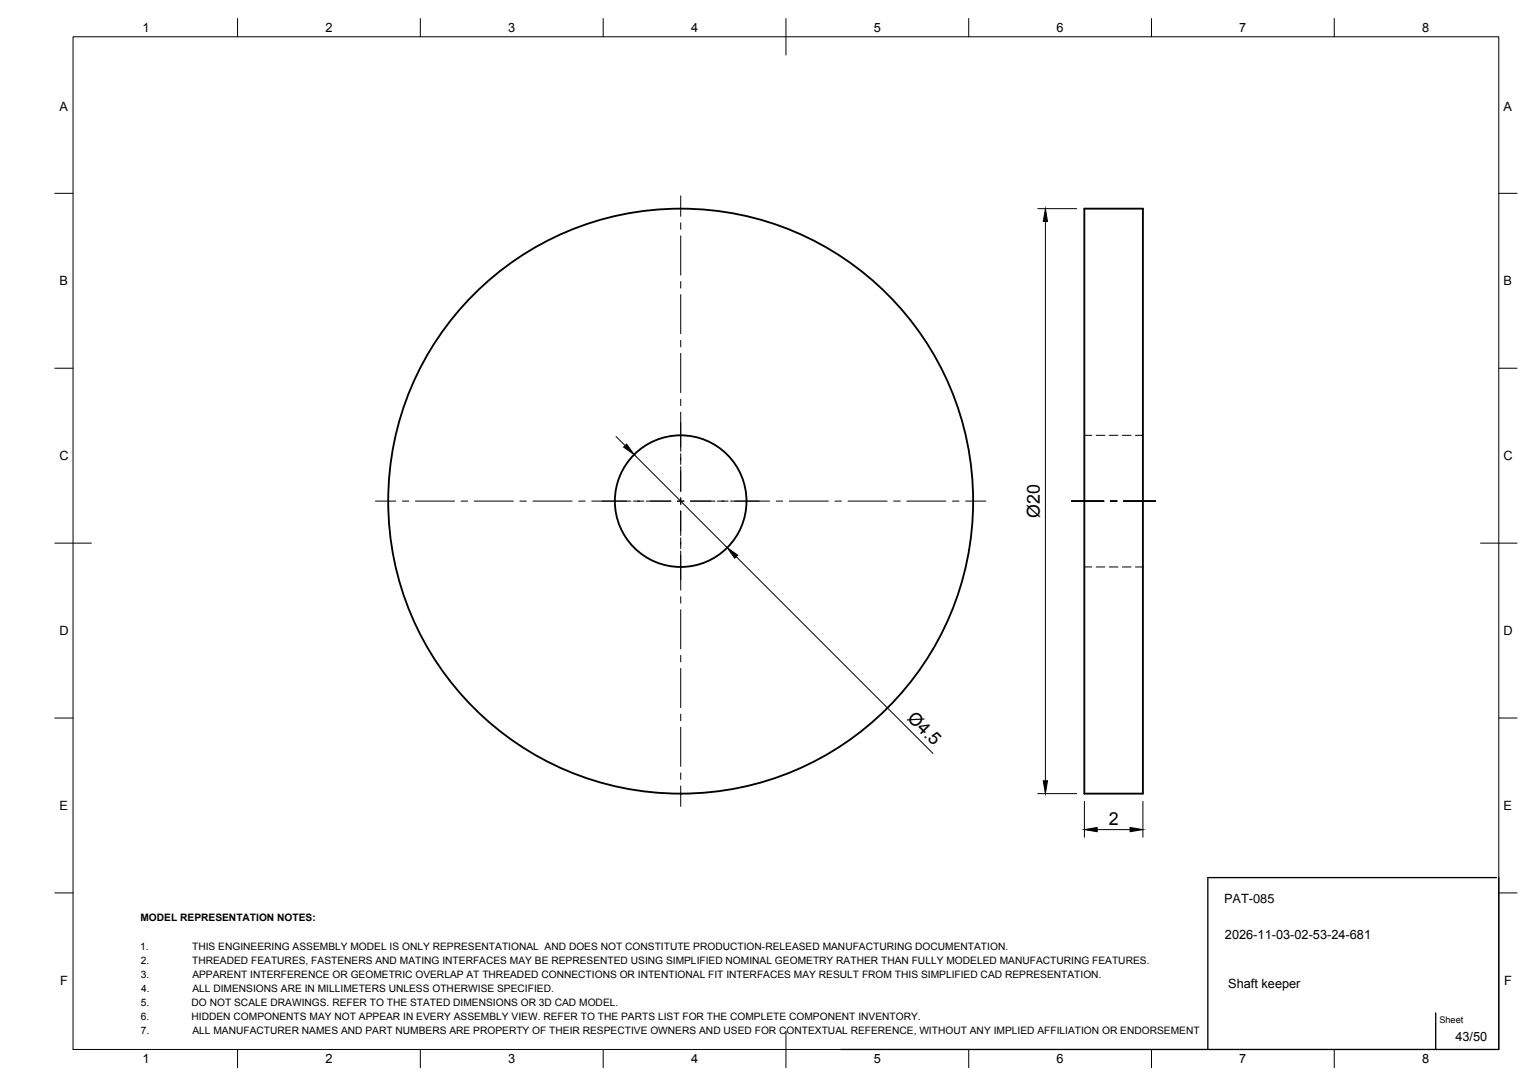
ISO-10303-21;
HEADER;
/* Generated by software containing ST-Developer
 * from STEP Tools, Inc. (www.steptools.com) 
 */

FILE_DESCRIPTION(
/* description */ ('Rack and pinion manual slide'),
/* implementation_level */ '2;1');

FILE_NAME(
/* name */ 'Shaft keeper.step',
/* time_stamp */ '2026-10-28T03:22:49-07:00',
/* author */ (''),
/* organization */ (''),
/* preprocessor_version */ 'ST-DEVELOPER v20.2',
/* originating_system */ 'Autodesk Translation Framework v15.17.0.0',
/* authorisation */ '');

FILE_SCHEMA (('AUTOMOTIVE_DESIGN { 1 0 10303 214 3 1 1 }'));
ENDSEC;

DATA;
#10=MECHANICAL_DESIGN_GEOMETRIC_PRESENTATION_REPRESENTATION('',(#774),#34851);
#675=SHAPE_REPRESENTATION_RELATIONSHIP('SRR','None',#35114,#721);
#721=ADVANCED_BREP_SHAPE_REPRESENTATION('',(#824),#34839);
#774=STYLED_ITEM('',(#35411),#824);
#824=MANIFOLD_SOLID_BREP('Body1',#13797);
#1022=FACE_BOUND('',#3036,.T.);
#1023=FACE_BOUND('',#3038,.T.);
#1456=PLANE('',#15269);
#1457=PLANE('',#15270);
#2105=FACE_OUTER_BOUND('',#3033,.T.);
#2106=FACE_OUTER_BOUND('',#3034,.T.);
#2107=FACE_OUTER_BOUND('',#3035,.T.);
#2108=FACE_OUTER_BOUND('',#3037,.T.);
#3033=EDGE_LOOP('',(#12026,#12027,#12028,#12029));
#3034=EDGE_LOOP('',(#12030,#12031,#12032,#12033));
#3035=EDGE_LOOP('',(#12034));
#3036=EDGE_LOOP('',(#12035));
#3037=EDGE_LOOP('',(#12036));
#3038=EDGE_LOOP('',(#12037));
#4280=LINE('',#22706,#5571);
#4281=LINE('',#22712,#5572);
#5571=VECTOR('',#18552,0.225);
#5572=VECTOR('',#18559,1.);
#6130=CIRCLE('',#15264,0.225);
#6131=CIRCLE('',#15265,0.225);
#6132=CIRCLE('',#15267,1.);
#6133=CIRCLE('',#15268,1.);
#7159=VERTEX_POINT('',#22703);
#7160=VERTEX_POINT('',#22705);
#7161=VERTEX_POINT('',#22709);
#7162=VERTEX_POINT('',#22711);
#8825=EDGE_CURVE('',#7159,#7159,#6130,.T.);
#8826=EDGE_CURVE('',#7159,#7160,#4280,.T.);
#8827=EDGE_CURVE('',#7160,#7160,#6131,.T.);
#8828=EDGE_CURVE('',#7161,#7161,#6132,.T.);
#8829=EDGE_CURVE('',#7161,#7162,#4281,.T.);
#8830=EDGE_CURVE('',#7162,#7162,#6133,.T.);
#12026=ORIENTED_EDGE('',*,*,#8825,.F.);
#12027=ORIENTED_EDGE('',*,*,#8826,.T.);
#12028=ORIENTED_EDGE('',*,*,#8827,.T.);
#12029=ORIENTED_EDGE('',*,*,#8826,.F.);
#12030=ORIENTED_EDGE('',*,*,#8828,.F.);
#12031=ORIENTED_EDGE('',*,*,#8829,.T.);
#12032=ORIENTED_EDGE('',*,*,#8830,.T.);
#12033=ORIENTED_EDGE('',*,*,#8829,.F.);
#12034=ORIENTED_EDGE('',*,*,#8828,.T.);
#12035=ORIENTED_EDGE('',*,*,#8825,.T.);
#12036=ORIENTED_EDGE('',*,*,#8830,.F.);
#12037=ORIENTED_EDGE('',*,*,#8827,.F.);
#12971=CYLINDRICAL_SURFACE('',#15263,0.225);
#12972=CYLINDRICAL_SURFACE('',#15266,1.);
#13583=ADVANCED_FACE('',(#2105),#12971,.F.);
#13584=ADVANCED_FACE('',(#2106),#12972,.T.);
#13585=ADVANCED_FACE('',(#2107,#1022),#1456,.T.);
#13586=ADVANCED_FACE('',(#2108,#1023),#1457,.F.);
#13797=CLOSED_SHELL('',(#13583,#13584,#13585,#13586));
#15262=AXIS2_PLACEMENT_3D('',#22701,#18546,#18547);
#15263=AXIS2_PLACEMENT_3D('',#22702,#18548,#18549);
#15264=AXIS2_PLACEMENT_3D('',#22704,#18550,#18551);
#15265=AXIS2_PLACEMENT_3D('',#22707,#18553,#18554);
#15266=AXIS2_PLACEMENT_3D('',#22708,#18555,#18556);
#15267=AXIS2_PLACEMENT_3D('',#22710,#18557,#18558);
#15268=AXIS2_PLACEMENT_3D('',#22713,#18560,#18561);
#15269=AXIS2_PLACEMENT_3D('',#22714,#18562,#18563);
#15270=AXIS2_PLACEMENT_3D('',#22715,#18564,#18565);
#18546=DIRECTION('axis',(0.,0.,1.));
#18547=DIRECTION('refdir',(1.,0.,0.));
#18548=DIRECTION('center_axis',(0.,1.,0.));
#18549=DIRECTION('ref_axis',(1.,0.,0.));
#18550=DIRECTION('center_axis',(0.,-1.,0.));
#18551=DIRECTION('ref_axis',(1.,0.,0.));
#18552=DIRECTION('',(0.,-1.,0.));
#18553=DIRECTION('center_axis',(0.,-1.,0.));
#18554=DIRECTION('ref_axis',(1.,0.,0.));
#18555=DIRECTION('center_axis',(0.,1.,0.));
#18556=DIRECTION('ref_axis',(1.,0.,0.));
#18557=DIRECTION('center_axis',(0.,1.,0.));
#18558=DIRECTION('ref_axis',(1.,0.,0.));
#18559=DIRECTION('',(0.,-1.,0.));
#18560=DIRECTION('center_axis',(0.,1.,0.));
#18561=DIRECTION('ref_axis',(1.,0.,0.));
#18562=DIRECTION('center_axis',(0.,1.,0.));
#18563=DIRECTION('ref_axis',(1.,0.,0.));
#18564=DIRECTION('center_axis',(0.,1.,0.));
#18565=DIRECTION('ref_axis',(1.,0.,0.));
#22701=CARTESIAN_POINT('',(0.,0.,0.));
#22702=CARTESIAN_POINT('Origin',(11.,-6.7,10.25));
#22703=CARTESIAN_POINT('',(10.775,-6.5,10.25));
#22704=CARTESIAN_POINT('Origin',(11.,-6.5,10.25));
#22705=CARTESIAN_POINT('',(10.775,-6.7,10.25));
#22706=CARTESIAN_POINT('',(10.775,-6.7,10.25));
#22707=CARTESIAN_POINT('Origin',(11.,-6.7,10.25));
#22708=CARTESIAN_POINT('Origin',(11.,-6.7,10.25));
#22709=CARTESIAN_POINT('',(10.,-6.5,10.25));
#22710=CARTESIAN_POINT('Origin',(11.,-6.5,10.25));
#22711=CARTESIAN_POINT('',(10.,-6.7,10.25));
#22712=CARTESIAN_POINT('',(10.,-6.7,10.25));
#22713=CARTESIAN_POINT('Origin',(11.,-6.7,10.25));
#22714=CARTESIAN_POINT('Origin',(11.,-6.5,10.25));
#22715=CARTESIAN_POINT('Origin',(11.,-6.7,10.25));
#34785=UNCERTAINTY_MEASURE_WITH_UNIT(LENGTH_MEASURE(0.001),#34852,
'DISTANCE_ACCURACY_VALUE',
'Maximum model space distance between geometric entities at asserted c
onnectivities');
#34797=UNCERTAINTY_MEASURE_WITH_UNIT(LENGTH_MEASURE(0.001),#34852,
'DISTANCE_ACCURACY_VALUE',
'Maximum model space distance between geometric entities at asserted c
onnectivities');
#34839=(
GEOMETRIC_REPRESENTATION_CONTEXT(3)
GLOBAL_UNCERTAINTY_ASSIGNED_CONTEXT((#34785))
GLOBAL_UNIT_ASSIGNED_CONTEXT((#34852,#34854,#34855))
REPRESENTATION_CONTEXT('','3D')
);
#34851=(
GEOMETRIC_REPRESENTATION_CONTEXT(3)
GLOBAL_UNCERTAINTY_ASSIGNED_CONTEXT((#34797))
GLOBAL_UNIT_ASSIGNED_CONTEXT((#34852,#34854,#34855))
REPRESENTATION_CONTEXT('','3D')
);
#34852=(
LENGTH_UNIT()
NAMED_UNIT(*)
SI_UNIT(.CENTI.,.METRE.)
);
#34854=(
NAMED_UNIT(*)
PLANE_ANGLE_UNIT()
SI_UNIT($,.RADIAN.)
);
#34855=(
NAMED_UNIT(*)
SI_UNIT($,.STERADIAN.)
SOLID_ANGLE_UNIT()
);
#34897=SHAPE_DEFINITION_REPRESENTATION(#34958,#35114);
#34958=PRODUCT_DEFINITION_SHAPE('',$,#35168);
#35114=SHAPE_REPRESENTATION('',(#15262),#34839);
#35126=PRODUCT_DEFINITION_CONTEXT('part definition',#35287,'design');
#35168=PRODUCT_DEFINITION('Shaft keeper','Shaft keeper',#35221,#35126);
#35221=PRODUCT_DEFINITION_FORMATION('',$,#35330);
#35287=APPLICATION_CONTEXT(
'Core Data for Automotive Mechanical Design Process');
#35288=PRODUCT_CONTEXT('part definition',#35287,'mechanical');
#35330=PRODUCT('Shaft keeper','Shaft keeper','Shaft keeper',(#35288));
#35405=COLOUR_RGB('Grey',0.48,0.52,0.57);
#35406=FILL_AREA_STYLE_COLOUR('',#35405);
#35407=FILL_AREA_STYLE('',(#35406));
#35408=SURFACE_STYLE_FILL_AREA(#35407);
#35409=SURFACE_SIDE_STYLE('',(#35408));
#35410=SURFACE_STYLE_USAGE(.BOTH.,#35409);
#35411=PRESENTATION_STYLE_ASSIGNMENT((#35410));
ENDSEC;
END-ISO-10303-21;
